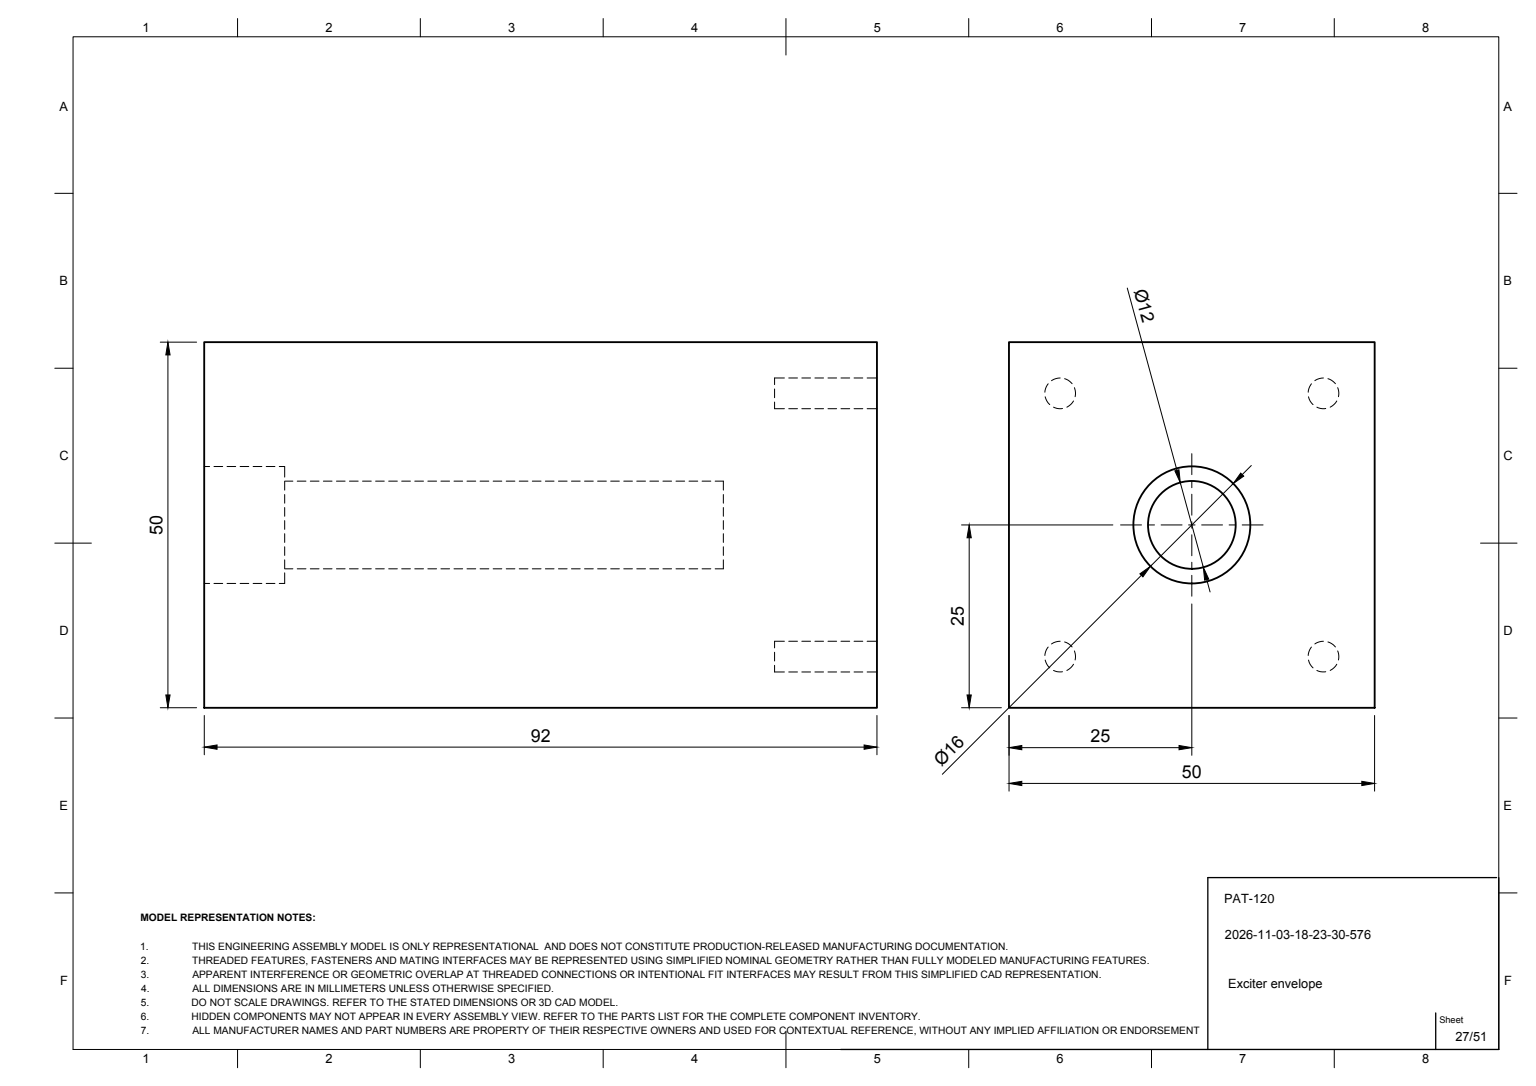
ISO-10303-21;
HEADER;
/* Generated by software containing ST-Developer
 * from STEP Tools, Inc. (www.steptools.com) 
 */

FILE_DESCRIPTION(
/* description */ ('Vibration shaker table dummy'),
/* implementation_level */ '2;1');

FILE_NAME(
/* name */ 'Exciter envelope.step',
/* time_stamp */ '2026-10-27T10:55:14-07:00',
/* author */ (''),
/* organization */ (''),
/* preprocessor_version */ 'ST-DEVELOPER v20.2',
/* originating_system */ 'Autodesk Translation Framework v15.17.0.0',
/* authorisation */ '');

FILE_SCHEMA (('AUTOMOTIVE_DESIGN { 1 0 10303 214 3 1 1 }'));
ENDSEC;

DATA;
#10=MECHANICAL_DESIGN_GEOMETRIC_PRESENTATION_REPRESENTATION('',(#708),#22394);
#616=SHAPE_REPRESENTATION_RELATIONSHIP('SRR','None',#22662,#662);
#662=ADVANCED_BREP_SHAPE_REPRESENTATION('',(#754),#22368);
#708=STYLED_ITEM('',(#22954),#754);
#754=MANIFOLD_SOLID_BREP('Body1',#9226);
#919=FACE_BOUND('',#2219,.T.);
#920=FACE_BOUND('',#2225,.T.);
#921=FACE_BOUND('',#2227,.T.);
#922=FACE_BOUND('',#2228,.T.);
#923=FACE_BOUND('',#2229,.T.);
#924=FACE_BOUND('',#2230,.T.);
#1192=PLANE('',#10208);
#1193=PLANE('',#10212);
#1194=PLANE('',#10216);
#1195=PLANE('',#10220);
#1196=PLANE('',#10224);
#1197=PLANE('',#10228);
#1198=PLANE('',#10229);
#1199=PLANE('',#10230);
#1200=PLANE('',#10231);
#1201=PLANE('',#10232);
#1202=PLANE('',#10233);
#1203=PLANE('',#10234);
#1565=FACE_OUTER_BOUND('',#2207,.T.);
#1566=FACE_OUTER_BOUND('',#2208,.T.);
#1567=FACE_OUTER_BOUND('',#2209,.T.);
#1568=FACE_OUTER_BOUND('',#2210,.T.);
#1569=FACE_OUTER_BOUND('',#2211,.T.);
#1570=FACE_OUTER_BOUND('',#2212,.T.);
#1571=FACE_OUTER_BOUND('',#2213,.T.);
#1572=FACE_OUTER_BOUND('',#2214,.T.);
#1573=FACE_OUTER_BOUND('',#2215,.T.);
#1574=FACE_OUTER_BOUND('',#2216,.T.);
#1575=FACE_OUTER_BOUND('',#2217,.T.);
#1576=FACE_OUTER_BOUND('',#2218,.T.);
#1577=FACE_OUTER_BOUND('',#2220,.T.);
#1578=FACE_OUTER_BOUND('',#2221,.T.);
#1579=FACE_OUTER_BOUND('',#2222,.T.);
#1580=FACE_OUTER_BOUND('',#2223,.T.);
#1581=FACE_OUTER_BOUND('',#2224,.T.);
#1582=FACE_OUTER_BOUND('',#2226,.T.);
#2207=EDGE_LOOP('',(#7278,#7279,#7280,#7281));
#2208=EDGE_LOOP('',(#7282));
#2209=EDGE_LOOP('',(#7283,#7284,#7285,#7286));
#2210=EDGE_LOOP('',(#7287));
#2211=EDGE_LOOP('',(#7288,#7289,#7290,#7291));
#2212=EDGE_LOOP('',(#7292));
#2213=EDGE_LOOP('',(#7293,#7294,#7295,#7296));
#2214=EDGE_LOOP('',(#7297));
#2215=EDGE_LOOP('',(#7298,#7299,#7300,#7301));
#2216=EDGE_LOOP('',(#7302));
#2217=EDGE_LOOP('',(#7303,#7304,#7305,#7306));
#2218=EDGE_LOOP('',(#7307));
#2219=EDGE_LOOP('',(#7308));
#2220=EDGE_LOOP('',(#7309,#7310,#7311,#7312));
#2221=EDGE_LOOP('',(#7313,#7314,#7315,#7316));
#2222=EDGE_LOOP('',(#7317,#7318,#7319,#7320));
#2223=EDGE_LOOP('',(#7321,#7322,#7323,#7324));
#2224=EDGE_LOOP('',(#7325,#7326,#7327,#7328));
#2225=EDGE_LOOP('',(#7329));
#2226=EDGE_LOOP('',(#7330,#7331,#7332,#7333));
#2227=EDGE_LOOP('',(#7334));
#2228=EDGE_LOOP('',(#7335));
#2229=EDGE_LOOP('',(#7336));
#2230=EDGE_LOOP('',(#7337));
#2934=LINE('',#20840,#3553);
#2935=LINE('',#20847,#3554);
#2936=LINE('',#20854,#3555);
#2937=LINE('',#20861,#3556);
#2938=LINE('',#20868,#3557);
#2939=LINE('',#20875,#3558);
#2940=LINE('',#20881,#3559);
#2941=LINE('',#20883,#3560);
#2942=LINE('',#20885,#3561);
#2943=LINE('',#20886,#3562);
#2944=LINE('',#20889,#3563);
#2945=LINE('',#20891,#3564);
#2946=LINE('',#20892,#3565);
#2947=LINE('',#20895,#3566);
#2948=LINE('',#20897,#3567);
#2949=LINE('',#20898,#3568);
#2950=LINE('',#20900,#3569);
#2951=LINE('',#20901,#3570);
#3553=VECTOR('',#12156,0.21);
#3554=VECTOR('',#12165,0.21);
#3555=VECTOR('',#12174,0.21);
#3556=VECTOR('',#12183,0.21);
#3557=VECTOR('',#12192,0.6);
#3558=VECTOR('',#12201,0.8);
#3559=VECTOR('',#12208,1.);
#3560=VECTOR('',#12209,1.);
#3561=VECTOR('',#12210,1.);
#3562=VECTOR('',#12211,1.);
#3563=VECTOR('',#12214,1.);
#3564=VECTOR('',#12215,1.);
#3565=VECTOR('',#12216,1.);
#3566=VECTOR('',#12219,1.);
#3567=VECTOR('',#12220,1.);
#3568=VECTOR('',#12221,1.);
#3569=VECTOR('',#12224,1.);
#3570=VECTOR('',#12225,1.);
#4060=CIRCLE('',#10206,0.21);
#4061=CIRCLE('',#10207,0.21);
#4062=CIRCLE('',#10210,0.21);
#4063=CIRCLE('',#10211,0.21);
#4064=CIRCLE('',#10214,0.21);
#4065=CIRCLE('',#10215,0.21);
#4066=CIRCLE('',#10218,0.21);
#4067=CIRCLE('',#10219,0.21);
#4068=CIRCLE('',#10222,0.6);
#4069=CIRCLE('',#10223,0.6);
#4070=CIRCLE('',#10226,0.8);
#4071=CIRCLE('',#10227,0.8);
#4711=VERTEX_POINT('',#20837);
#4712=VERTEX_POINT('',#20839);
#4713=VERTEX_POINT('',#20844);
#4714=VERTEX_POINT('',#20846);
#4715=VERTEX_POINT('',#20851);
#4716=VERTEX_POINT('',#20853);
#4717=VERTEX_POINT('',#20858);
#4718=VERTEX_POINT('',#20860);
#4719=VERTEX_POINT('',#20865);
#4720=VERTEX_POINT('',#20867);
#4721=VERTEX_POINT('',#20872);
#4722=VERTEX_POINT('',#20874);
#4723=VERTEX_POINT('',#20879);
#4724=VERTEX_POINT('',#20880);
#4725=VERTEX_POINT('',#20882);
#4726=VERTEX_POINT('',#20884);
#4727=VERTEX_POINT('',#20888);
#4728=VERTEX_POINT('',#20890);
#4729=VERTEX_POINT('',#20894);
#4730=VERTEX_POINT('',#20896);
#5632=EDGE_CURVE('',#4711,#4711,#4060,.T.);
#5633=EDGE_CURVE('',#4711,#4712,#2934,.T.);
#5634=EDGE_CURVE('',#4712,#4712,#4061,.T.);
#5635=EDGE_CURVE('',#4713,#4713,#4062,.T.);
#5636=EDGE_CURVE('',#4713,#4714,#2935,.T.);
#5637=EDGE_CURVE('',#4714,#4714,#4063,.T.);
#5638=EDGE_CURVE('',#4715,#4715,#4064,.T.);
#5639=EDGE_CURVE('',#4715,#4716,#2936,.T.);
#5640=EDGE_CURVE('',#4716,#4716,#4065,.T.);
#5641=EDGE_CURVE('',#4717,#4717,#4066,.T.);
#5642=EDGE_CURVE('',#4717,#4718,#2937,.T.);
#5643=EDGE_CURVE('',#4718,#4718,#4067,.T.);
#5644=EDGE_CURVE('',#4719,#4719,#4068,.T.);
#5645=EDGE_CURVE('',#4719,#4720,#2938,.T.);
#5646=EDGE_CURVE('',#4720,#4720,#4069,.T.);
#5647=EDGE_CURVE('',#4721,#4721,#4070,.T.);
#5648=EDGE_CURVE('',#4721,#4722,#2939,.T.);
#5649=EDGE_CURVE('',#4722,#4722,#4071,.T.);
#5650=EDGE_CURVE('',#4723,#4724,#2940,.T.);
#5651=EDGE_CURVE('',#4724,#4725,#2941,.T.);
#5652=EDGE_CURVE('',#4726,#4725,#2942,.T.);
#5653=EDGE_CURVE('',#4723,#4726,#2943,.T.);
#5654=EDGE_CURVE('',#4727,#4723,#2944,.T.);
#5655=EDGE_CURVE('',#4728,#4726,#2945,.T.);
#5656=EDGE_CURVE('',#4727,#4728,#2946,.T.);
#5657=EDGE_CURVE('',#4729,#4727,#2947,.T.);
#5658=EDGE_CURVE('',#4730,#4728,#2948,.T.);
#5659=EDGE_CURVE('',#4729,#4730,#2949,.T.);
#5660=EDGE_CURVE('',#4724,#4729,#2950,.T.);
#5661=EDGE_CURVE('',#4725,#4730,#2951,.T.);
#7278=ORIENTED_EDGE('',*,*,#5632,.F.);
#7279=ORIENTED_EDGE('',*,*,#5633,.T.);
#7280=ORIENTED_EDGE('',*,*,#5634,.T.);
#7281=ORIENTED_EDGE('',*,*,#5633,.F.);
#7282=ORIENTED_EDGE('',*,*,#5634,.F.);
#7283=ORIENTED_EDGE('',*,*,#5635,.F.);
#7284=ORIENTED_EDGE('',*,*,#5636,.T.);
#7285=ORIENTED_EDGE('',*,*,#5637,.T.);
#7286=ORIENTED_EDGE('',*,*,#5636,.F.);
#7287=ORIENTED_EDGE('',*,*,#5637,.F.);
#7288=ORIENTED_EDGE('',*,*,#5638,.F.);
#7289=ORIENTED_EDGE('',*,*,#5639,.T.);
#7290=ORIENTED_EDGE('',*,*,#5640,.T.);
#7291=ORIENTED_EDGE('',*,*,#5639,.F.);
#7292=ORIENTED_EDGE('',*,*,#5640,.F.);
#7293=ORIENTED_EDGE('',*,*,#5641,.F.);
#7294=ORIENTED_EDGE('',*,*,#5642,.T.);
#7295=ORIENTED_EDGE('',*,*,#5643,.T.);
#7296=ORIENTED_EDGE('',*,*,#5642,.F.);
#7297=ORIENTED_EDGE('',*,*,#5643,.F.);
#7298=ORIENTED_EDGE('',*,*,#5644,.F.);
#7299=ORIENTED_EDGE('',*,*,#5645,.T.);
#7300=ORIENTED_EDGE('',*,*,#5646,.F.);
#7301=ORIENTED_EDGE('',*,*,#5645,.F.);
#7302=ORIENTED_EDGE('',*,*,#5644,.T.);
#7303=ORIENTED_EDGE('',*,*,#5647,.F.);
#7304=ORIENTED_EDGE('',*,*,#5648,.T.);
#7305=ORIENTED_EDGE('',*,*,#5649,.F.);
#7306=ORIENTED_EDGE('',*,*,#5648,.F.);
#7307=ORIENTED_EDGE('',*,*,#5647,.T.);
#7308=ORIENTED_EDGE('',*,*,#5646,.T.);
#7309=ORIENTED_EDGE('',*,*,#5650,.T.);
#7310=ORIENTED_EDGE('',*,*,#5651,.T.);
#7311=ORIENTED_EDGE('',*,*,#5652,.F.);
#7312=ORIENTED_EDGE('',*,*,#5653,.F.);
#7313=ORIENTED_EDGE('',*,*,#5654,.T.);
#7314=ORIENTED_EDGE('',*,*,#5653,.T.);
#7315=ORIENTED_EDGE('',*,*,#5655,.F.);
#7316=ORIENTED_EDGE('',*,*,#5656,.F.);
#7317=ORIENTED_EDGE('',*,*,#5657,.T.);
#7318=ORIENTED_EDGE('',*,*,#5656,.T.);
#7319=ORIENTED_EDGE('',*,*,#5658,.F.);
#7320=ORIENTED_EDGE('',*,*,#5659,.F.);
#7321=ORIENTED_EDGE('',*,*,#5660,.T.);
#7322=ORIENTED_EDGE('',*,*,#5659,.T.);
#7323=ORIENTED_EDGE('',*,*,#5661,.F.);
#7324=ORIENTED_EDGE('',*,*,#5651,.F.);
#7325=ORIENTED_EDGE('',*,*,#5661,.T.);
#7326=ORIENTED_EDGE('',*,*,#5658,.T.);
#7327=ORIENTED_EDGE('',*,*,#5655,.T.);
#7328=ORIENTED_EDGE('',*,*,#5652,.T.);
#7329=ORIENTED_EDGE('',*,*,#5649,.T.);
#7330=ORIENTED_EDGE('',*,*,#5660,.F.);
#7331=ORIENTED_EDGE('',*,*,#5650,.F.);
#7332=ORIENTED_EDGE('',*,*,#5654,.F.);
#7333=ORIENTED_EDGE('',*,*,#5657,.F.);
#7334=ORIENTED_EDGE('',*,*,#5632,.T.);
#7335=ORIENTED_EDGE('',*,*,#5635,.T.);
#7336=ORIENTED_EDGE('',*,*,#5638,.T.);
#7337=ORIENTED_EDGE('',*,*,#5641,.T.);
#8594=CYLINDRICAL_SURFACE('',#10205,0.21);
#8595=CYLINDRICAL_SURFACE('',#10209,0.21);
#8596=CYLINDRICAL_SURFACE('',#10213,0.21);
#8597=CYLINDRICAL_SURFACE('',#10217,0.21);
#8598=CYLINDRICAL_SURFACE('',#10221,0.6);
#8599=CYLINDRICAL_SURFACE('',#10225,0.8);
#8930=ADVANCED_FACE('',(#1565),#8594,.F.);
#8931=ADVANCED_FACE('',(#1566),#1192,.F.);
#8932=ADVANCED_FACE('',(#1567),#8595,.F.);
#8933=ADVANCED_FACE('',(#1568),#1193,.F.);
#8934=ADVANCED_FACE('',(#1569),#8596,.F.);
#8935=ADVANCED_FACE('',(#1570),#1194,.F.);
#8936=ADVANCED_FACE('',(#1571),#8597,.F.);
#8937=ADVANCED_FACE('',(#1572),#1195,.F.);
#8938=ADVANCED_FACE('',(#1573),#8598,.F.);
#8939=ADVANCED_FACE('',(#1574),#1196,.T.);
#8940=ADVANCED_FACE('',(#1575),#8599,.F.);
#8941=ADVANCED_FACE('',(#1576,#919),#1197,.T.);
#8942=ADVANCED_FACE('',(#1577),#1198,.T.);
#8943=ADVANCED_FACE('',(#1578),#1199,.T.);
#8944=ADVANCED_FACE('',(#1579),#1200,.T.);
#8945=ADVANCED_FACE('',(#1580),#1201,.T.);
#8946=ADVANCED_FACE('',(#1581,#920),#1202,.T.);
#8947=ADVANCED_FACE('',(#1582,#921,#922,#923,#924),#1203,.F.);
#9226=CLOSED_SHELL('',(#8930,#8931,#8932,#8933,#8934,#8935,#8936,#8937,
#8938,#8939,#8940,#8941,#8942,#8943,#8944,#8945,#8946,#8947));
#10204=AXIS2_PLACEMENT_3D('',#20835,#12150,#12151);
#10205=AXIS2_PLACEMENT_3D('',#20836,#12152,#12153);
#10206=AXIS2_PLACEMENT_3D('',#20838,#12154,#12155);
#10207=AXIS2_PLACEMENT_3D('',#20841,#12157,#12158);
#10208=AXIS2_PLACEMENT_3D('',#20842,#12159,#12160);
#10209=AXIS2_PLACEMENT_3D('',#20843,#12161,#12162);
#10210=AXIS2_PLACEMENT_3D('',#20845,#12163,#12164);
#10211=AXIS2_PLACEMENT_3D('',#20848,#12166,#12167);
#10212=AXIS2_PLACEMENT_3D('',#20849,#12168,#12169);
#10213=AXIS2_PLACEMENT_3D('',#20850,#12170,#12171);
#10214=AXIS2_PLACEMENT_3D('',#20852,#12172,#12173);
#10215=AXIS2_PLACEMENT_3D('',#20855,#12175,#12176);
#10216=AXIS2_PLACEMENT_3D('',#20856,#12177,#12178);
#10217=AXIS2_PLACEMENT_3D('',#20857,#12179,#12180);
#10218=AXIS2_PLACEMENT_3D('',#20859,#12181,#12182);
#10219=AXIS2_PLACEMENT_3D('',#20862,#12184,#12185);
#10220=AXIS2_PLACEMENT_3D('',#20863,#12186,#12187);
#10221=AXIS2_PLACEMENT_3D('',#20864,#12188,#12189);
#10222=AXIS2_PLACEMENT_3D('',#20866,#12190,#12191);
#10223=AXIS2_PLACEMENT_3D('',#20869,#12193,#12194);
#10224=AXIS2_PLACEMENT_3D('',#20870,#12195,#12196);
#10225=AXIS2_PLACEMENT_3D('',#20871,#12197,#12198);
#10226=AXIS2_PLACEMENT_3D('',#20873,#12199,#12200);
#10227=AXIS2_PLACEMENT_3D('',#20876,#12202,#12203);
#10228=AXIS2_PLACEMENT_3D('',#20877,#12204,#12205);
#10229=AXIS2_PLACEMENT_3D('',#20878,#12206,#12207);
#10230=AXIS2_PLACEMENT_3D('',#20887,#12212,#12213);
#10231=AXIS2_PLACEMENT_3D('',#20893,#12217,#12218);
#10232=AXIS2_PLACEMENT_3D('',#20899,#12222,#12223);
#10233=AXIS2_PLACEMENT_3D('',#20902,#12226,#12227);
#10234=AXIS2_PLACEMENT_3D('',#20903,#12228,#12229);
#12150=DIRECTION('axis',(0.,0.,1.));
#12151=DIRECTION('refdir',(1.,0.,0.));
#12152=DIRECTION('center_axis',(0.,0.,1.));
#12153=DIRECTION('ref_axis',(1.,0.,0.));
#12154=DIRECTION('center_axis',(0.,0.,1.));
#12155=DIRECTION('ref_axis',(1.,0.,0.));
#12156=DIRECTION('',(0.,0.,1.));
#12157=DIRECTION('center_axis',(0.,0.,1.));
#12158=DIRECTION('ref_axis',(1.,0.,0.));
#12159=DIRECTION('center_axis',(0.,0.,1.));
#12160=DIRECTION('ref_axis',(1.,0.,0.));
#12161=DIRECTION('center_axis',(0.,0.,1.));
#12162=DIRECTION('ref_axis',(1.,0.,0.));
#12163=DIRECTION('center_axis',(0.,0.,1.));
#12164=DIRECTION('ref_axis',(1.,0.,0.));
#12165=DIRECTION('',(0.,0.,1.));
#12166=DIRECTION('center_axis',(0.,0.,1.));
#12167=DIRECTION('ref_axis',(1.,0.,0.));
#12168=DIRECTION('center_axis',(0.,0.,1.));
#12169=DIRECTION('ref_axis',(1.,0.,0.));
#12170=DIRECTION('center_axis',(0.,0.,1.));
#12171=DIRECTION('ref_axis',(1.,0.,0.));
#12172=DIRECTION('center_axis',(0.,0.,1.));
#12173=DIRECTION('ref_axis',(1.,0.,0.));
#12174=DIRECTION('',(0.,0.,1.));
#12175=DIRECTION('center_axis',(0.,0.,1.));
#12176=DIRECTION('ref_axis',(1.,0.,0.));
#12177=DIRECTION('center_axis',(0.,0.,1.));
#12178=DIRECTION('ref_axis',(1.,0.,0.));
#12179=DIRECTION('center_axis',(0.,0.,1.));
#12180=DIRECTION('ref_axis',(1.,0.,0.));
#12181=DIRECTION('center_axis',(0.,0.,1.));
#12182=DIRECTION('ref_axis',(1.,0.,0.));
#12183=DIRECTION('',(0.,0.,1.));
#12184=DIRECTION('center_axis',(0.,0.,1.));
#12185=DIRECTION('ref_axis',(1.,0.,0.));
#12186=DIRECTION('center_axis',(0.,0.,1.));
#12187=DIRECTION('ref_axis',(1.,0.,0.));
#12188=DIRECTION('center_axis',(0.,0.,1.));
#12189=DIRECTION('ref_axis',(1.,0.,0.));
#12190=DIRECTION('center_axis',(0.,0.,1.));
#12191=DIRECTION('ref_axis',(1.,0.,0.));
#12192=DIRECTION('',(0.,0.,1.));
#12193=DIRECTION('center_axis',(0.,0.,-1.));
#12194=DIRECTION('ref_axis',(1.,0.,0.));
#12195=DIRECTION('center_axis',(0.,0.,1.));
#12196=DIRECTION('ref_axis',(1.,0.,0.));
#12197=DIRECTION('center_axis',(0.,0.,1.));
#12198=DIRECTION('ref_axis',(1.,0.,0.));
#12199=DIRECTION('center_axis',(0.,0.,1.));
#12200=DIRECTION('ref_axis',(1.,0.,0.));
#12201=DIRECTION('',(0.,0.,1.));
#12202=DIRECTION('center_axis',(0.,0.,-1.));
#12203=DIRECTION('ref_axis',(1.,0.,0.));
#12204=DIRECTION('center_axis',(0.,0.,1.));
#12205=DIRECTION('ref_axis',(1.,0.,0.));
#12206=DIRECTION('center_axis',(0.,1.,0.));
#12207=DIRECTION('ref_axis',(-1.,0.,0.));
#12208=DIRECTION('',(-1.,0.,0.));
#12209=DIRECTION('',(0.,0.,1.));
#12210=DIRECTION('',(-1.,0.,0.));
#12211=DIRECTION('',(0.,0.,1.));
#12212=DIRECTION('center_axis',(1.,0.,0.));
#12213=DIRECTION('ref_axis',(0.,1.,0.));
#12214=DIRECTION('',(0.,1.,0.));
#12215=DIRECTION('',(0.,1.,0.));
#12216=DIRECTION('',(0.,0.,1.));
#12217=DIRECTION('center_axis',(0.,-1.,0.));
#12218=DIRECTION('ref_axis',(1.,0.,0.));
#12219=DIRECTION('',(1.,0.,0.));
#12220=DIRECTION('',(1.,0.,0.));
#12221=DIRECTION('',(0.,0.,1.));
#12222=DIRECTION('center_axis',(-1.,0.,0.));
#12223=DIRECTION('ref_axis',(0.,-1.,0.));
#12224=DIRECTION('',(0.,-1.,0.));
#12225=DIRECTION('',(0.,-1.,0.));
#12226=DIRECTION('center_axis',(0.,0.,1.));
#12227=DIRECTION('ref_axis',(1.,0.,0.));
#12228=DIRECTION('center_axis',(0.,0.,1.));
#12229=DIRECTION('ref_axis',(1.,0.,0.));
#20835=CARTESIAN_POINT('',(0.,0.,0.));
#20836=CARTESIAN_POINT('Origin',(1.8,-1.8,0.7));
#20837=CARTESIAN_POINT('',(1.59,-1.8,0.8));
#20838=CARTESIAN_POINT('Origin',(1.8,-1.8,0.8));
#20839=CARTESIAN_POINT('',(1.59,-1.8,2.2));
#20840=CARTESIAN_POINT('',(1.59,-1.8,0.7));
#20841=CARTESIAN_POINT('Origin',(1.8,-1.8,2.2));
#20842=CARTESIAN_POINT('Origin',(1.8,-1.8,2.2));
#20843=CARTESIAN_POINT('Origin',(-1.8,1.8,0.7));
#20844=CARTESIAN_POINT('',(-2.01,1.8,0.8));
#20845=CARTESIAN_POINT('Origin',(-1.8,1.8,0.8));
#20846=CARTESIAN_POINT('',(-2.01,1.8,2.2));
#20847=CARTESIAN_POINT('',(-2.01,1.8,0.7));
#20848=CARTESIAN_POINT('Origin',(-1.8,1.8,2.2));
#20849=CARTESIAN_POINT('Origin',(-1.8,1.8,2.2));
#20850=CARTESIAN_POINT('Origin',(-1.8,-1.8,0.7));
#20851=CARTESIAN_POINT('',(-2.01,-1.8,0.8));
#20852=CARTESIAN_POINT('Origin',(-1.8,-1.8,0.8));
#20853=CARTESIAN_POINT('',(-2.01,-1.8,2.2));
#20854=CARTESIAN_POINT('',(-2.01,-1.8,0.7));
#20855=CARTESIAN_POINT('Origin',(-1.8,-1.8,2.2));
#20856=CARTESIAN_POINT('Origin',(-1.8,-1.8,2.2));
#20857=CARTESIAN_POINT('Origin',(1.8,1.8,0.7));
#20858=CARTESIAN_POINT('',(1.59,1.8,0.8));
#20859=CARTESIAN_POINT('Origin',(1.8,1.8,0.8));
#20860=CARTESIAN_POINT('',(1.59,1.8,2.2));
#20861=CARTESIAN_POINT('',(1.59,1.8,0.7));
#20862=CARTESIAN_POINT('Origin',(1.8,1.8,2.2));
#20863=CARTESIAN_POINT('Origin',(1.8,1.8,2.2));
#20864=CARTESIAN_POINT('Origin',(0.,0.,2.9));
#20865=CARTESIAN_POINT('',(-0.6,-7.34788079488412E-17,2.9));
#20866=CARTESIAN_POINT('Origin',(0.,0.,2.9));
#20867=CARTESIAN_POINT('',(-0.6,7.34788079488412E-17,8.9));
#20868=CARTESIAN_POINT('',(-0.6,-7.34788079488412E-17,2.9));
#20869=CARTESIAN_POINT('Origin',(0.,0.,8.9));
#20870=CARTESIAN_POINT('Origin',(0.,0.,2.9));
#20871=CARTESIAN_POINT('Origin',(0.,0.,8.9));
#20872=CARTESIAN_POINT('',(-0.8,-9.79717439317883E-17,8.9));
#20873=CARTESIAN_POINT('Origin',(0.,0.,8.9));
#20874=CARTESIAN_POINT('',(-0.8,9.79717439317883E-17,10.));
#20875=CARTESIAN_POINT('',(-0.8,-9.79717439317883E-17,8.9));
#20876=CARTESIAN_POINT('Origin',(0.,0.,10.));
#20877=CARTESIAN_POINT('Origin',(0.,0.,8.9));
#20878=CARTESIAN_POINT('Origin',(2.5,2.5,0.8));
#20879=CARTESIAN_POINT('',(2.5,2.5,0.8));
#20880=CARTESIAN_POINT('',(-2.5,2.5,0.8));
#20881=CARTESIAN_POINT('',(2.5,2.5,0.8));
#20882=CARTESIAN_POINT('',(-2.5,2.5,10.));
#20883=CARTESIAN_POINT('',(-2.5,2.5,0.8));
#20884=CARTESIAN_POINT('',(2.5,2.5,10.));
#20885=CARTESIAN_POINT('',(2.5,2.5,10.));
#20886=CARTESIAN_POINT('',(2.5,2.5,0.8));
#20887=CARTESIAN_POINT('Origin',(2.5,-2.5,0.8));
#20888=CARTESIAN_POINT('',(2.5,-2.5,0.8));
#20889=CARTESIAN_POINT('',(2.5,-2.5,0.8));
#20890=CARTESIAN_POINT('',(2.5,-2.5,10.));
#20891=CARTESIAN_POINT('',(2.5,-2.5,10.));
#20892=CARTESIAN_POINT('',(2.5,-2.5,0.8));
#20893=CARTESIAN_POINT('Origin',(-2.5,-2.5,0.8));
#20894=CARTESIAN_POINT('',(-2.5,-2.5,0.8));
#20895=CARTESIAN_POINT('',(-2.5,-2.5,0.8));
#20896=CARTESIAN_POINT('',(-2.5,-2.5,10.));
#20897=CARTESIAN_POINT('',(-2.5,-2.5,10.));
#20898=CARTESIAN_POINT('',(-2.5,-2.5,0.8));
#20899=CARTESIAN_POINT('Origin',(-2.5,2.5,0.8));
#20900=CARTESIAN_POINT('',(-2.5,2.5,0.8));
#20901=CARTESIAN_POINT('',(-2.5,2.5,10.));
#20902=CARTESIAN_POINT('Origin',(0.,0.,10.));
#20903=CARTESIAN_POINT('Origin',(0.,0.,0.8));
#22317=UNCERTAINTY_MEASURE_WITH_UNIT(LENGTH_MEASURE(0.001),#22395,
'DISTANCE_ACCURACY_VALUE',
'Maximum model space distance between geometric entities at asserted c
onnectivities');
#22343=UNCERTAINTY_MEASURE_WITH_UNIT(LENGTH_MEASURE(0.001),#22395,
'DISTANCE_ACCURACY_VALUE',
'Maximum model space distance between geometric entities at asserted c
onnectivities');
#22368=(
GEOMETRIC_REPRESENTATION_CONTEXT(3)
GLOBAL_UNCERTAINTY_ASSIGNED_CONTEXT((#22317))
GLOBAL_UNIT_ASSIGNED_CONTEXT((#22395,#22397,#22398))
REPRESENTATION_CONTEXT('','3D')
);
#22394=(
GEOMETRIC_REPRESENTATION_CONTEXT(3)
GLOBAL_UNCERTAINTY_ASSIGNED_CONTEXT((#22343))
GLOBAL_UNIT_ASSIGNED_CONTEXT((#22395,#22397,#22398))
REPRESENTATION_CONTEXT('','3D')
);
#22395=(
LENGTH_UNIT()
NAMED_UNIT(*)
SI_UNIT(.CENTI.,.METRE.)
);
#22397=(
NAMED_UNIT(*)
PLANE_ANGLE_UNIT()
SI_UNIT($,.RADIAN.)
);
#22398=(
NAMED_UNIT(*)
SI_UNIT($,.STERADIAN.)
SOLID_ANGLE_UNIT()
);
#22423=SHAPE_DEFINITION_REPRESENTATION(#22473,#22662);
#22473=PRODUCT_DEFINITION_SHAPE('',$,#22713);
#22662=SHAPE_REPRESENTATION('',(#10204),#22368);
#22688=PRODUCT_DEFINITION_CONTEXT('part definition',#22840,'design');
#22713=PRODUCT_DEFINITION('Exciter envelope','Exciter envelope',#22763,
#22688);
#22763=PRODUCT_DEFINITION_FORMATION('',$,#22866);
#22840=APPLICATION_CONTEXT(
'Core Data for Automotive Mechanical Design Process');
#22841=PRODUCT_CONTEXT('part definition',#22840,'mechanical');
#22866=PRODUCT('Exciter envelope','Exciter envelope','Exciter envelope',
(#22841));
#22948=COLOUR_RGB('Sky Blue',0.24,0.69,0.87);
#22949=FILL_AREA_STYLE_COLOUR('',#22948);
#22950=FILL_AREA_STYLE('',(#22949));
#22951=SURFACE_STYLE_FILL_AREA(#22950);
#22952=SURFACE_SIDE_STYLE('',(#22951));
#22953=SURFACE_STYLE_USAGE(.BOTH.,#22952);
#22954=PRESENTATION_STYLE_ASSIGNMENT((#22953));
ENDSEC;
END-ISO-10303-21;
